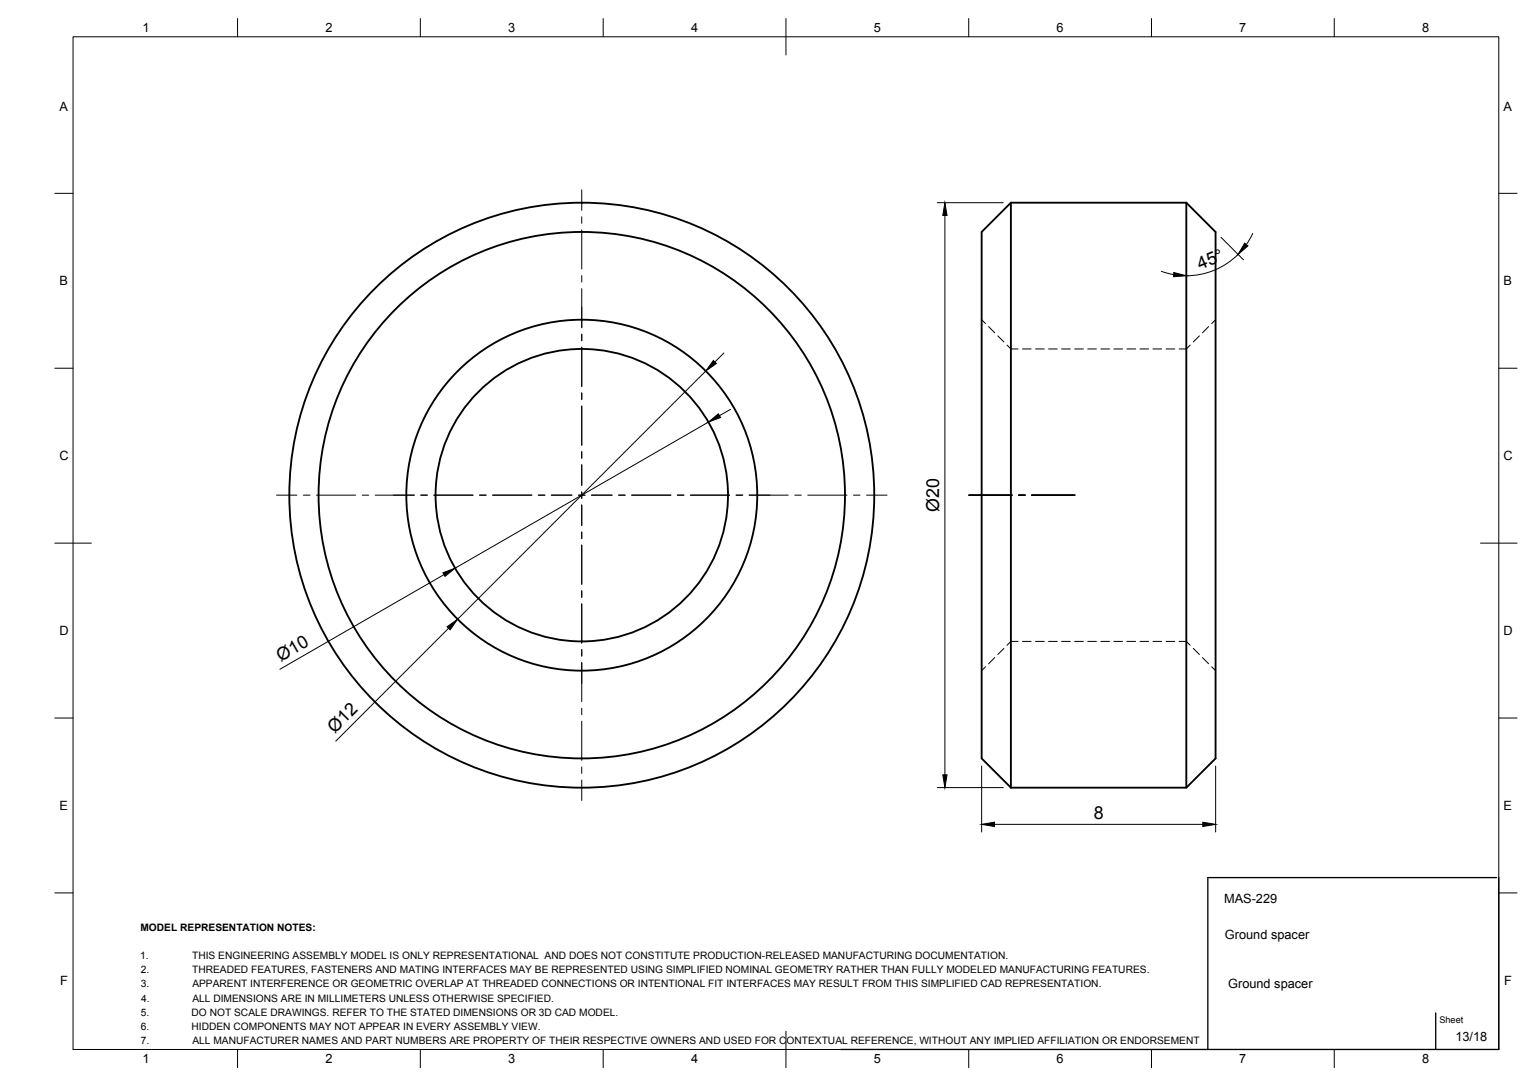
ISO-10303-21;
HEADER;
/* Generated by software containing ST-Developer
 * from STEP Tools, Inc. (www.steptools.com) 
 */

FILE_DESCRIPTION(
/* description */ ('Independently dimensioned six-bar single-leg walking-linkage demonstr
ator. Whole-mm20 crank,60 upper rocker,80/120 ternary coupler,120 lowe
r rocker,140 knee pitch and260 toe reach; ground pivots0/0,60/0,40/60.
 Seven native revolutes close both loops. Four reused native library f
amilies, fully retained shared pins and layered real spacer stacks, bo
nded rubber toe. Benchtop reference mechanism; no complete vehicle, lo
ad, gait stability, adhesive, weld, fit or life rating.'),
/* implementation_level */ '2;1');

FILE_NAME(
/* name */ 'Ground spacer.step',
/* time_stamp */ '2026-11-09T20:33:14-08:00',
/* author */ (''),
/* organization */ (''),
/* preprocessor_version */ 'ST-DEVELOPER v20.2',
/* originating_system */ 'Autodesk Translation Framework v15.17.0.0',
/* authorisation */ '');

FILE_SCHEMA (('AUTOMOTIVE_DESIGN { 1 0 10303 214 3 1 1 }'));
ENDSEC;

DATA;
#10=MECHANICAL_DESIGN_GEOMETRIC_PRESENTATION_REPRESENTATION('',(#265),#4048);
#215=CONICAL_SURFACE('',#2521,9.5,0.785398163397448);
#216=CONICAL_SURFACE('',#2528,9.5,0.785398163397448);
#217=CONICAL_SURFACE('',#2532,5.5,0.785398163397448);
#218=CONICAL_SURFACE('',#2536,5.5,0.785398163397448);
#229=SHAPE_REPRESENTATION_RELATIONSHIP('SRR','None',#4153,#247);
#247=ADVANCED_BREP_SHAPE_REPRESENTATION('',(#283),#4040);
#265=STYLED_ITEM('',(#4241),#283);
#283=MANIFOLD_SOLID_BREP('Spacer',#2154);
#332=FACE_BOUND('',#663,.T.);
#333=FACE_BOUND('',#666,.T.);
#391=PLANE('',#2526);
#392=PLANE('',#2530);
#493=FACE_OUTER_BOUND('',#660,.T.);
#494=FACE_OUTER_BOUND('',#661,.T.);
#495=FACE_OUTER_BOUND('',#662,.T.);
#496=FACE_OUTER_BOUND('',#664,.T.);
#497=FACE_OUTER_BOUND('',#665,.T.);
#498=FACE_OUTER_BOUND('',#667,.T.);
#499=FACE_OUTER_BOUND('',#668,.T.);
#500=FACE_OUTER_BOUND('',#669,.T.);
#660=EDGE_LOOP('',(#1815,#1816,#1817,#1818));
#661=EDGE_LOOP('',(#1819,#1820,#1821,#1822));
#662=EDGE_LOOP('',(#1823));
#663=EDGE_LOOP('',(#1824));
#664=EDGE_LOOP('',(#1825,#1826,#1827,#1828));
#665=EDGE_LOOP('',(#1829));
#666=EDGE_LOOP('',(#1830));
#667=EDGE_LOOP('',(#1831,#1832,#1833,#1834));
#668=EDGE_LOOP('',(#1835,#1836,#1837,#1838));
#669=EDGE_LOOP('',(#1839,#1840,#1841,#1842));
#819=LINE('',#3785,#944);
#820=LINE('',#3790,#945);
#821=LINE('',#3797,#946);
#822=LINE('',#3804,#947);
#823=LINE('',#3808,#948);
#824=LINE('',#3810,#949);
#944=VECTOR('',#3090,9.5);
#945=VECTOR('',#3097,10.);
#946=VECTOR('',#3106,9.5);
#947=VECTOR('',#3115,5.5);
#948=VECTOR('',#3120,5.);
#949=VECTOR('',#3123,5.5);
#1044=CIRCLE('',#2522,10.);
#1045=CIRCLE('',#2523,9.);
#1046=CIRCLE('',#2525,10.);
#1047=CIRCLE('',#2527,6.);
#1048=CIRCLE('',#2529,9.);
#1049=CIRCLE('',#2531,6.);
#1050=CIRCLE('',#2533,5.);
#1051=CIRCLE('',#2535,5.);
#1198=VERTEX_POINT('',#3782);
#1199=VERTEX_POINT('',#3784);
#1200=VERTEX_POINT('',#3788);
#1201=VERTEX_POINT('',#3792);
#1202=VERTEX_POINT('',#3795);
#1203=VERTEX_POINT('',#3799);
#1204=VERTEX_POINT('',#3802);
#1205=VERTEX_POINT('',#3806);
#1411=EDGE_CURVE('',#1198,#1198,#1044,.T.);
#1412=EDGE_CURVE('',#1198,#1199,#819,.T.);
#1413=EDGE_CURVE('',#1199,#1199,#1045,.T.);
#1414=EDGE_CURVE('',#1200,#1200,#1046,.T.);
#1415=EDGE_CURVE('',#1200,#1198,#820,.T.);
#1416=EDGE_CURVE('',#1201,#1201,#1047,.T.);
#1417=EDGE_CURVE('',#1202,#1202,#1048,.T.);
#1418=EDGE_CURVE('',#1202,#1200,#821,.T.);
#1419=EDGE_CURVE('',#1203,#1203,#1049,.T.);
#1420=EDGE_CURVE('',#1204,#1204,#1050,.T.);
#1421=EDGE_CURVE('',#1204,#1201,#822,.T.);
#1422=EDGE_CURVE('',#1205,#1205,#1051,.T.);
#1423=EDGE_CURVE('',#1205,#1204,#823,.T.);
#1424=EDGE_CURVE('',#1203,#1205,#824,.T.);
#1815=ORIENTED_EDGE('',*,*,#1411,.T.);
#1816=ORIENTED_EDGE('',*,*,#1412,.T.);
#1817=ORIENTED_EDGE('',*,*,#1413,.T.);
#1818=ORIENTED_EDGE('',*,*,#1412,.F.);
#1819=ORIENTED_EDGE('',*,*,#1414,.F.);
#1820=ORIENTED_EDGE('',*,*,#1415,.T.);
#1821=ORIENTED_EDGE('',*,*,#1411,.F.);
#1822=ORIENTED_EDGE('',*,*,#1415,.F.);
#1823=ORIENTED_EDGE('',*,*,#1413,.F.);
#1824=ORIENTED_EDGE('',*,*,#1416,.F.);
#1825=ORIENTED_EDGE('',*,*,#1417,.T.);
#1826=ORIENTED_EDGE('',*,*,#1418,.T.);
#1827=ORIENTED_EDGE('',*,*,#1414,.T.);
#1828=ORIENTED_EDGE('',*,*,#1418,.F.);
#1829=ORIENTED_EDGE('',*,*,#1417,.F.);
#1830=ORIENTED_EDGE('',*,*,#1419,.F.);
#1831=ORIENTED_EDGE('',*,*,#1420,.T.);
#1832=ORIENTED_EDGE('',*,*,#1421,.T.);
#1833=ORIENTED_EDGE('',*,*,#1416,.T.);
#1834=ORIENTED_EDGE('',*,*,#1421,.F.);
#1835=ORIENTED_EDGE('',*,*,#1422,.F.);
#1836=ORIENTED_EDGE('',*,*,#1423,.T.);
#1837=ORIENTED_EDGE('',*,*,#1420,.F.);
#1838=ORIENTED_EDGE('',*,*,#1423,.F.);
#1839=ORIENTED_EDGE('',*,*,#1419,.T.);
#1840=ORIENTED_EDGE('',*,*,#1424,.T.);
#1841=ORIENTED_EDGE('',*,*,#1422,.T.);
#1842=ORIENTED_EDGE('',*,*,#1424,.F.);
#1998=CYLINDRICAL_SURFACE('',#2524,10.);
#1999=CYLINDRICAL_SURFACE('',#2534,5.);
#2096=ADVANCED_FACE('',(#493),#215,.T.);
#2097=ADVANCED_FACE('',(#494),#1998,.T.);
#2098=ADVANCED_FACE('',(#495,#332),#391,.F.);
#2099=ADVANCED_FACE('',(#496),#216,.T.);
#2100=ADVANCED_FACE('',(#497,#333),#392,.T.);
#2101=ADVANCED_FACE('',(#498),#217,.F.);
#2102=ADVANCED_FACE('',(#499),#1999,.F.);
#2103=ADVANCED_FACE('',(#500),#218,.F.);
#2154=CLOSED_SHELL('',(#2096,#2097,#2098,#2099,#2100,#2101,#2102,#2103));
#2520=AXIS2_PLACEMENT_3D('',#3780,#3084,#3085);
#2521=AXIS2_PLACEMENT_3D('',#3781,#3086,#3087);
#2522=AXIS2_PLACEMENT_3D('',#3783,#3088,#3089);
#2523=AXIS2_PLACEMENT_3D('',#3786,#3091,#3092);
#2524=AXIS2_PLACEMENT_3D('',#3787,#3093,#3094);
#2525=AXIS2_PLACEMENT_3D('',#3789,#3095,#3096);
#2526=AXIS2_PLACEMENT_3D('',#3791,#3098,#3099);
#2527=AXIS2_PLACEMENT_3D('',#3793,#3100,#3101);
#2528=AXIS2_PLACEMENT_3D('',#3794,#3102,#3103);
#2529=AXIS2_PLACEMENT_3D('',#3796,#3104,#3105);
#2530=AXIS2_PLACEMENT_3D('',#3798,#3107,#3108);
#2531=AXIS2_PLACEMENT_3D('',#3800,#3109,#3110);
#2532=AXIS2_PLACEMENT_3D('',#3801,#3111,#3112);
#2533=AXIS2_PLACEMENT_3D('',#3803,#3113,#3114);
#2534=AXIS2_PLACEMENT_3D('',#3805,#3116,#3117);
#2535=AXIS2_PLACEMENT_3D('',#3807,#3118,#3119);
#2536=AXIS2_PLACEMENT_3D('',#3809,#3121,#3122);
#3084=DIRECTION('axis',(0.,0.,1.));
#3085=DIRECTION('refdir',(1.,0.,0.));
#3086=DIRECTION('center_axis',(0.,0.,1.));
#3087=DIRECTION('ref_axis',(1.,0.,0.));
#3088=DIRECTION('center_axis',(0.,0.,-1.));
#3089=DIRECTION('ref_axis',(1.,0.,0.));
#3090=DIRECTION('',(0.707106781186547,8.65956056235493E-17,-0.707106781186548));
#3091=DIRECTION('center_axis',(0.,0.,1.));
#3092=DIRECTION('ref_axis',(1.,0.,0.));
#3093=DIRECTION('center_axis',(0.,0.,1.));
#3094=DIRECTION('ref_axis',(1.,0.,0.));
#3095=DIRECTION('center_axis',(0.,0.,1.));
#3096=DIRECTION('ref_axis',(1.,0.,0.));
#3097=DIRECTION('',(0.,0.,-1.));
#3098=DIRECTION('center_axis',(0.,0.,1.));
#3099=DIRECTION('ref_axis',(1.,0.,0.));
#3100=DIRECTION('center_axis',(0.,0.,-1.));
#3101=DIRECTION('ref_axis',(1.,0.,0.));
#3102=DIRECTION('center_axis',(0.,0.,-1.));
#3103=DIRECTION('ref_axis',(1.,0.,0.));
#3104=DIRECTION('center_axis',(0.,0.,-1.));
#3105=DIRECTION('ref_axis',(1.,0.,0.));
#3106=DIRECTION('',(-0.707106781186548,-8.65956056235493E-17,-0.707106781186548));
#3107=DIRECTION('center_axis',(0.,0.,1.));
#3108=DIRECTION('ref_axis',(1.,0.,0.));
#3109=DIRECTION('center_axis',(0.,0.,1.));
#3110=DIRECTION('ref_axis',(1.,0.,0.));
#3111=DIRECTION('center_axis',(0.,0.,-1.));
#3112=DIRECTION('ref_axis',(1.,0.,0.));
#3113=DIRECTION('center_axis',(0.,0.,1.));
#3114=DIRECTION('ref_axis',(1.,0.,0.));
#3115=DIRECTION('',(-0.707106781186547,-8.65956056235493E-17,-0.707106781186548));
#3116=DIRECTION('center_axis',(0.,0.,1.));
#3117=DIRECTION('ref_axis',(1.,0.,0.));
#3118=DIRECTION('center_axis',(0.,0.,-1.));
#3119=DIRECTION('ref_axis',(1.,0.,0.));
#3120=DIRECTION('',(0.,0.,-1.));
#3121=DIRECTION('center_axis',(0.,0.,1.));
#3122=DIRECTION('ref_axis',(1.,0.,0.));
#3123=DIRECTION('',(0.707106781186548,8.65956056235493E-17,-0.707106781186548));
#3780=CARTESIAN_POINT('',(0.,0.,0.));
#3781=CARTESIAN_POINT('Origin',(0.,0.,0.5));
#3782=CARTESIAN_POINT('',(-10.,1.22464679914735E-15,1.));
#3783=CARTESIAN_POINT('Origin',(0.,0.,1.));
#3784=CARTESIAN_POINT('',(-9.,-1.10218211923262E-15,0.));
#3785=CARTESIAN_POINT('',(-9.5,-1.16341445918999E-15,0.5));
#3786=CARTESIAN_POINT('Origin',(0.,0.,0.));
#3787=CARTESIAN_POINT('Origin',(0.,0.,0.));
#3788=CARTESIAN_POINT('',(-10.,-1.22464679914735E-15,7.));
#3789=CARTESIAN_POINT('Origin',(0.,0.,7.));
#3790=CARTESIAN_POINT('',(-10.,-1.22464679914735E-15,0.));
#3791=CARTESIAN_POINT('Origin',(0.,0.,0.));
#3792=CARTESIAN_POINT('',(-6.,7.34788079488412E-16,0.));
#3793=CARTESIAN_POINT('Origin',(0.,0.,0.));
#3794=CARTESIAN_POINT('Origin',(0.,0.,7.5));
#3795=CARTESIAN_POINT('',(-9.,1.10218211923262E-15,8.));
#3796=CARTESIAN_POINT('Origin',(0.,0.,8.));
#3797=CARTESIAN_POINT('',(-9.5,-1.16341445918999E-15,7.5));
#3798=CARTESIAN_POINT('Origin',(0.,0.,8.));
#3799=CARTESIAN_POINT('',(-6.,-7.34788079488412E-16,8.));
#3800=CARTESIAN_POINT('Origin',(0.,0.,8.));
#3801=CARTESIAN_POINT('Origin',(0.,0.,0.5));
#3802=CARTESIAN_POINT('',(-5.,-6.12323399573677E-16,1.));
#3803=CARTESIAN_POINT('Origin',(0.,0.,1.));
#3804=CARTESIAN_POINT('',(-5.5,-6.73555739531044E-16,0.5));
#3805=CARTESIAN_POINT('Origin',(0.,0.,0.));
#3806=CARTESIAN_POINT('',(-5.,6.12323399573677E-16,7.));
#3807=CARTESIAN_POINT('Origin',(0.,0.,7.));
#3808=CARTESIAN_POINT('',(-5.,-6.12323399573677E-16,0.));
#3809=CARTESIAN_POINT('Origin',(0.,0.,7.5));
#3810=CARTESIAN_POINT('',(-5.5,-6.73555739531044E-16,7.5));
#4020=UNCERTAINTY_MEASURE_WITH_UNIT(LENGTH_MEASURE(0.01),#4049,
'DISTANCE_ACCURACY_VALUE',
'Maximum model space distance between geometric entities at asserted c
onnectivities');
#4028=UNCERTAINTY_MEASURE_WITH_UNIT(LENGTH_MEASURE(0.01),#4049,
'DISTANCE_ACCURACY_VALUE',
'Maximum model space distance between geometric entities at asserted c
onnectivities');
#4040=(
GEOMETRIC_REPRESENTATION_CONTEXT(3)
GLOBAL_UNCERTAINTY_ASSIGNED_CONTEXT((#4020))
GLOBAL_UNIT_ASSIGNED_CONTEXT((#4049,#4051,#4052))
REPRESENTATION_CONTEXT('','3D')
);
#4048=(
GEOMETRIC_REPRESENTATION_CONTEXT(3)
GLOBAL_UNCERTAINTY_ASSIGNED_CONTEXT((#4028))
GLOBAL_UNIT_ASSIGNED_CONTEXT((#4049,#4051,#4052))
REPRESENTATION_CONTEXT('','3D')
);
#4049=(
LENGTH_UNIT()
NAMED_UNIT(*)
SI_UNIT(.MILLI.,.METRE.)
);
#4051=(
NAMED_UNIT(*)
PLANE_ANGLE_UNIT()
SI_UNIT($,.RADIAN.)
);
#4052=(
NAMED_UNIT(*)
SI_UNIT($,.STERADIAN.)
SOLID_ANGLE_UNIT()
);
#4064=SHAPE_DEFINITION_REPRESENTATION(#4083,#4153);
#4083=PRODUCT_DEFINITION_SHAPE('',$,#4173);
#4153=SHAPE_REPRESENTATION('',(#2520),#4040);
#4161=PRODUCT_DEFINITION_CONTEXT('part definition',#4220,'design');
#4173=PRODUCT_DEFINITION('Ground spacer','Ground spacer',#4192,#4161);
#4192=PRODUCT_DEFINITION_FORMATION('',$,#4233);
#4220=APPLICATION_CONTEXT(
'Core Data for Automotive Mechanical Design Process');
#4221=PRODUCT_CONTEXT('part definition',#4220,'mechanical');
#4233=PRODUCT('Ground spacer','Ground spacer',
'Turn OD, drill bore, face to length. Nominal dimensions in mm. Fit li
mits to be assigned at assembly level.',(#4221));
#4241=PRESENTATION_STYLE_ASSIGNMENT((#4255));
#4255=SURFACE_STYLE_USAGE(.BOTH.,#4269);
#4269=SURFACE_SIDE_STYLE('',(#4283));
#4283=SURFACE_STYLE_FILL_AREA(#4297);
#4297=FILL_AREA_STYLE('Steel - Satin',(#4311));
#4311=FILL_AREA_STYLE_COLOUR('Steel - Satin',#4325);
#4325=COLOUR_RGB('Steel - Satin',0.627450980392157,0.627450980392157,0.627450980392157);
ENDSEC;
END-ISO-10303-21;
